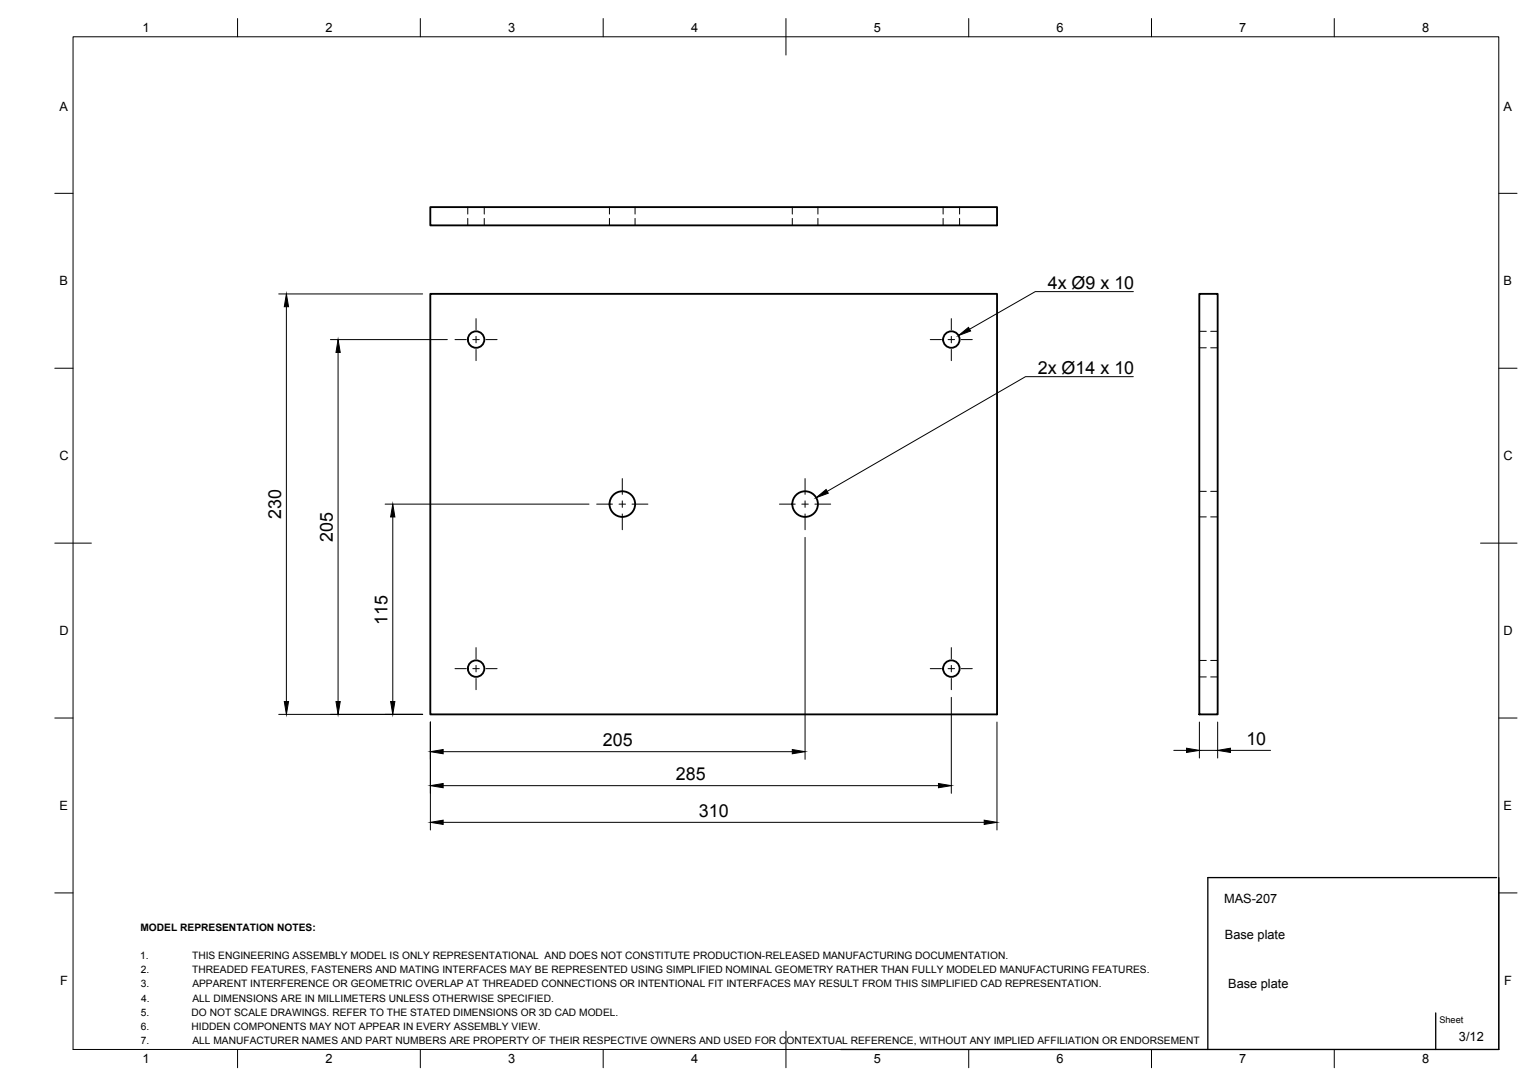
ISO-10303-21;
HEADER;
/* Generated by software containing ST-Developer
 * from STEP Tools, Inc. (www.steptools.com) 
 */

FILE_DESCRIPTION(
/* description */ ('Independent six-slot Geneva indexer. Center distance100, drive radius
50, 60degree indexing per input revolution with120degree engagement an
d240degree dwell. Native machined concave locking faces and relieved d
isk; replaceable retained drive pin; keyed output shaft. Geometry traj
ectory checks use calculated indexing positions, not a contact-dynamic
s simulation. No load or production rating assigned.'),
/* implementation_level */ '2;1');

FILE_NAME(
/* name */ 'Base plate.step',
/* time_stamp */ '2026-11-09T17:53:22-08:00',
/* author */ (''),
/* organization */ (''),
/* preprocessor_version */ 'ST-DEVELOPER v20.2',
/* originating_system */ 'Autodesk Translation Framework v15.17.0.0',
/* authorisation */ '');

FILE_SCHEMA (('AUTOMOTIVE_DESIGN { 1 0 10303 214 3 1 1 }'));
ENDSEC;

DATA;
#10=MECHANICAL_DESIGN_GEOMETRIC_PRESENTATION_REPRESENTATION('',(#101),#4149);
#79=SHAPE_REPRESENTATION_RELATIONSHIP('SRR','None',#4196,#90);
#90=ADVANCED_BREP_SHAPE_REPRESENTATION('',(#112),#4138);
#101=STYLED_ITEM('',(#4260),#112);
#112=MANIFOLD_SOLID_BREP('Body1',#2295);
#123=FACE_BOUND('',#385,.T.);
#124=FACE_BOUND('',#386,.T.);
#125=FACE_BOUND('',#387,.T.);
#126=FACE_BOUND('',#388,.T.);
#127=FACE_BOUND('',#389,.T.);
#128=FACE_BOUND('',#390,.T.);
#129=FACE_BOUND('',#392,.T.);
#130=FACE_BOUND('',#393,.T.);
#131=FACE_BOUND('',#394,.T.);
#132=FACE_BOUND('',#395,.T.);
#133=FACE_BOUND('',#396,.T.);
#134=FACE_BOUND('',#397,.T.);
#161=PLANE('',#2448);
#162=PLANE('',#2449);
#163=PLANE('',#2450);
#164=PLANE('',#2451);
#165=PLANE('',#2452);
#166=PLANE('',#2453);
#238=FACE_OUTER_BOUND('',#374,.T.);
#239=FACE_OUTER_BOUND('',#375,.T.);
#240=FACE_OUTER_BOUND('',#376,.T.);
#241=FACE_OUTER_BOUND('',#377,.T.);
#242=FACE_OUTER_BOUND('',#378,.T.);
#243=FACE_OUTER_BOUND('',#379,.T.);
#244=FACE_OUTER_BOUND('',#380,.T.);
#245=FACE_OUTER_BOUND('',#381,.T.);
#246=FACE_OUTER_BOUND('',#382,.T.);
#247=FACE_OUTER_BOUND('',#383,.T.);
#248=FACE_OUTER_BOUND('',#384,.T.);
#249=FACE_OUTER_BOUND('',#391,.T.);
#374=EDGE_LOOP('',(#1508,#1509,#1510,#1511));
#375=EDGE_LOOP('',(#1512,#1513,#1514,#1515));
#376=EDGE_LOOP('',(#1516,#1517,#1518,#1519));
#377=EDGE_LOOP('',(#1520,#1521,#1522,#1523));
#378=EDGE_LOOP('',(#1524,#1525,#1526,#1527));
#379=EDGE_LOOP('',(#1528,#1529,#1530,#1531));
#380=EDGE_LOOP('',(#1532,#1533,#1534,#1535));
#381=EDGE_LOOP('',(#1536,#1537,#1538,#1539));
#382=EDGE_LOOP('',(#1540,#1541,#1542,#1543));
#383=EDGE_LOOP('',(#1544,#1545,#1546,#1547));
#384=EDGE_LOOP('',(#1548,#1549,#1550,#1551));
#385=EDGE_LOOP('',(#1552));
#386=EDGE_LOOP('',(#1553));
#387=EDGE_LOOP('',(#1554));
#388=EDGE_LOOP('',(#1555));
#389=EDGE_LOOP('',(#1556));
#390=EDGE_LOOP('',(#1557));
#391=EDGE_LOOP('',(#1558,#1559,#1560,#1561));
#392=EDGE_LOOP('',(#1562));
#393=EDGE_LOOP('',(#1563));
#394=EDGE_LOOP('',(#1564));
#395=EDGE_LOOP('',(#1565));
#396=EDGE_LOOP('',(#1566));
#397=EDGE_LOOP('',(#1567));
#548=LINE('',#3473,#720);
#549=LINE('',#3479,#721);
#550=LINE('',#3485,#722);
#551=LINE('',#3491,#723);
#552=LINE('',#3497,#724);
#553=LINE('',#3503,#725);
#554=LINE('',#3508,#726);
#555=LINE('',#3510,#727);
#556=LINE('',#3512,#728);
#557=LINE('',#3513,#729);
#558=LINE('',#3516,#730);
#559=LINE('',#3518,#731);
#560=LINE('',#3519,#732);
#561=LINE('',#3522,#733);
#562=LINE('',#3524,#734);
#563=LINE('',#3525,#735);
#564=LINE('',#3527,#736);
#565=LINE('',#3528,#737);
#720=VECTOR('',#2725,4.5);
#721=VECTOR('',#2732,4.5);
#722=VECTOR('',#2739,4.5);
#723=VECTOR('',#2746,4.5);
#724=VECTOR('',#2753,7.);
#725=VECTOR('',#2760,7.);
#726=VECTOR('',#2765,10.);
#727=VECTOR('',#2766,10.);
#728=VECTOR('',#2767,10.);
#729=VECTOR('',#2768,10.);
#730=VECTOR('',#2771,10.);
#731=VECTOR('',#2772,10.);
#732=VECTOR('',#2773,10.);
#733=VECTOR('',#2776,10.);
#734=VECTOR('',#2777,10.);
#735=VECTOR('',#2778,10.);
#736=VECTOR('',#2781,10.);
#737=VECTOR('',#2782,10.);
#892=CIRCLE('',#2431,4.5);
#893=CIRCLE('',#2432,4.5);
#894=CIRCLE('',#2434,4.5);
#895=CIRCLE('',#2435,4.5);
#896=CIRCLE('',#2437,4.5);
#897=CIRCLE('',#2438,4.5);
#898=CIRCLE('',#2440,4.5);
#899=CIRCLE('',#2441,4.5);
#900=CIRCLE('',#2443,7.);
#901=CIRCLE('',#2444,7.);
#902=CIRCLE('',#2446,7.);
#903=CIRCLE('',#2447,7.);
#1016=VERTEX_POINT('',#3470);
#1017=VERTEX_POINT('',#3472);
#1018=VERTEX_POINT('',#3476);
#1019=VERTEX_POINT('',#3478);
#1020=VERTEX_POINT('',#3482);
#1021=VERTEX_POINT('',#3484);
#1022=VERTEX_POINT('',#3488);
#1023=VERTEX_POINT('',#3490);
#1024=VERTEX_POINT('',#3494);
#1025=VERTEX_POINT('',#3496);
#1026=VERTEX_POINT('',#3500);
#1027=VERTEX_POINT('',#3502);
#1028=VERTEX_POINT('',#3506);
#1029=VERTEX_POINT('',#3507);
#1030=VERTEX_POINT('',#3509);
#1031=VERTEX_POINT('',#3511);
#1032=VERTEX_POINT('',#3515);
#1033=VERTEX_POINT('',#3517);
#1034=VERTEX_POINT('',#3521);
#1035=VERTEX_POINT('',#3523);
#1212=EDGE_CURVE('',#1016,#1016,#892,.T.);
#1213=EDGE_CURVE('',#1016,#1017,#548,.T.);
#1214=EDGE_CURVE('',#1017,#1017,#893,.T.);
#1215=EDGE_CURVE('',#1018,#1018,#894,.T.);
#1216=EDGE_CURVE('',#1018,#1019,#549,.T.);
#1217=EDGE_CURVE('',#1019,#1019,#895,.T.);
#1218=EDGE_CURVE('',#1020,#1020,#896,.T.);
#1219=EDGE_CURVE('',#1020,#1021,#550,.T.);
#1220=EDGE_CURVE('',#1021,#1021,#897,.T.);
#1221=EDGE_CURVE('',#1022,#1022,#898,.T.);
#1222=EDGE_CURVE('',#1022,#1023,#551,.T.);
#1223=EDGE_CURVE('',#1023,#1023,#899,.T.);
#1224=EDGE_CURVE('',#1024,#1024,#900,.T.);
#1225=EDGE_CURVE('',#1024,#1025,#552,.T.);
#1226=EDGE_CURVE('',#1025,#1025,#901,.T.);
#1227=EDGE_CURVE('',#1026,#1026,#902,.T.);
#1228=EDGE_CURVE('',#1026,#1027,#553,.T.);
#1229=EDGE_CURVE('',#1027,#1027,#903,.T.);
#1230=EDGE_CURVE('',#1028,#1029,#554,.F.);
#1231=EDGE_CURVE('',#1029,#1030,#555,.F.);
#1232=EDGE_CURVE('',#1031,#1030,#556,.F.);
#1233=EDGE_CURVE('',#1028,#1031,#557,.F.);
#1234=EDGE_CURVE('',#1032,#1028,#558,.F.);
#1235=EDGE_CURVE('',#1033,#1031,#559,.F.);
#1236=EDGE_CURVE('',#1032,#1033,#560,.F.);
#1237=EDGE_CURVE('',#1034,#1032,#561,.F.);
#1238=EDGE_CURVE('',#1035,#1033,#562,.F.);
#1239=EDGE_CURVE('',#1034,#1035,#563,.T.);
#1240=EDGE_CURVE('',#1029,#1034,#564,.F.);
#1241=EDGE_CURVE('',#1030,#1035,#565,.F.);
#1508=ORIENTED_EDGE('',*,*,#1212,.F.);
#1509=ORIENTED_EDGE('',*,*,#1213,.T.);
#1510=ORIENTED_EDGE('',*,*,#1214,.F.);
#1511=ORIENTED_EDGE('',*,*,#1213,.F.);
#1512=ORIENTED_EDGE('',*,*,#1215,.F.);
#1513=ORIENTED_EDGE('',*,*,#1216,.T.);
#1514=ORIENTED_EDGE('',*,*,#1217,.F.);
#1515=ORIENTED_EDGE('',*,*,#1216,.F.);
#1516=ORIENTED_EDGE('',*,*,#1218,.F.);
#1517=ORIENTED_EDGE('',*,*,#1219,.T.);
#1518=ORIENTED_EDGE('',*,*,#1220,.F.);
#1519=ORIENTED_EDGE('',*,*,#1219,.F.);
#1520=ORIENTED_EDGE('',*,*,#1221,.F.);
#1521=ORIENTED_EDGE('',*,*,#1222,.T.);
#1522=ORIENTED_EDGE('',*,*,#1223,.F.);
#1523=ORIENTED_EDGE('',*,*,#1222,.F.);
#1524=ORIENTED_EDGE('',*,*,#1224,.F.);
#1525=ORIENTED_EDGE('',*,*,#1225,.T.);
#1526=ORIENTED_EDGE('',*,*,#1226,.F.);
#1527=ORIENTED_EDGE('',*,*,#1225,.F.);
#1528=ORIENTED_EDGE('',*,*,#1227,.F.);
#1529=ORIENTED_EDGE('',*,*,#1228,.T.);
#1530=ORIENTED_EDGE('',*,*,#1229,.F.);
#1531=ORIENTED_EDGE('',*,*,#1228,.F.);
#1532=ORIENTED_EDGE('',*,*,#1230,.T.);
#1533=ORIENTED_EDGE('',*,*,#1231,.T.);
#1534=ORIENTED_EDGE('',*,*,#1232,.F.);
#1535=ORIENTED_EDGE('',*,*,#1233,.F.);
#1536=ORIENTED_EDGE('',*,*,#1234,.T.);
#1537=ORIENTED_EDGE('',*,*,#1233,.T.);
#1538=ORIENTED_EDGE('',*,*,#1235,.F.);
#1539=ORIENTED_EDGE('',*,*,#1236,.F.);
#1540=ORIENTED_EDGE('',*,*,#1237,.T.);
#1541=ORIENTED_EDGE('',*,*,#1236,.T.);
#1542=ORIENTED_EDGE('',*,*,#1238,.F.);
#1543=ORIENTED_EDGE('',*,*,#1239,.F.);
#1544=ORIENTED_EDGE('',*,*,#1240,.T.);
#1545=ORIENTED_EDGE('',*,*,#1239,.T.);
#1546=ORIENTED_EDGE('',*,*,#1241,.F.);
#1547=ORIENTED_EDGE('',*,*,#1231,.F.);
#1548=ORIENTED_EDGE('',*,*,#1241,.T.);
#1549=ORIENTED_EDGE('',*,*,#1238,.T.);
#1550=ORIENTED_EDGE('',*,*,#1235,.T.);
#1551=ORIENTED_EDGE('',*,*,#1232,.T.);
#1552=ORIENTED_EDGE('',*,*,#1227,.T.);
#1553=ORIENTED_EDGE('',*,*,#1224,.T.);
#1554=ORIENTED_EDGE('',*,*,#1221,.T.);
#1555=ORIENTED_EDGE('',*,*,#1218,.T.);
#1556=ORIENTED_EDGE('',*,*,#1215,.T.);
#1557=ORIENTED_EDGE('',*,*,#1212,.T.);
#1558=ORIENTED_EDGE('',*,*,#1240,.F.);
#1559=ORIENTED_EDGE('',*,*,#1230,.F.);
#1560=ORIENTED_EDGE('',*,*,#1234,.F.);
#1561=ORIENTED_EDGE('',*,*,#1237,.F.);
#1562=ORIENTED_EDGE('',*,*,#1229,.T.);
#1563=ORIENTED_EDGE('',*,*,#1226,.T.);
#1564=ORIENTED_EDGE('',*,*,#1223,.T.);
#1565=ORIENTED_EDGE('',*,*,#1220,.T.);
#1566=ORIENTED_EDGE('',*,*,#1217,.T.);
#1567=ORIENTED_EDGE('',*,*,#1214,.T.);
#2100=CYLINDRICAL_SURFACE('',#2430,4.5);
#2101=CYLINDRICAL_SURFACE('',#2433,4.5);
#2102=CYLINDRICAL_SURFACE('',#2436,4.5);
#2103=CYLINDRICAL_SURFACE('',#2439,4.5);
#2104=CYLINDRICAL_SURFACE('',#2442,7.);
#2105=CYLINDRICAL_SURFACE('',#2445,7.);
#2159=ADVANCED_FACE('',(#238),#2100,.F.);
#2160=ADVANCED_FACE('',(#239),#2101,.F.);
#2161=ADVANCED_FACE('',(#240),#2102,.F.);
#2162=ADVANCED_FACE('',(#241),#2103,.F.);
#2163=ADVANCED_FACE('',(#242),#2104,.F.);
#2164=ADVANCED_FACE('',(#243),#2105,.F.);
#2165=ADVANCED_FACE('',(#244),#161,.T.);
#2166=ADVANCED_FACE('',(#245),#162,.T.);
#2167=ADVANCED_FACE('',(#246),#163,.T.);
#2168=ADVANCED_FACE('',(#247),#164,.T.);
#2169=ADVANCED_FACE('',(#248,#123,#124,#125,#126,#127,#128),#165,.T.);
#2170=ADVANCED_FACE('',(#249,#129,#130,#131,#132,#133,#134),#166,.F.);
#2295=CLOSED_SHELL('',(#2159,#2160,#2161,#2162,#2163,#2164,#2165,#2166,
#2167,#2168,#2169,#2170));
#2429=AXIS2_PLACEMENT_3D('',#3468,#2719,#2720);
#2430=AXIS2_PLACEMENT_3D('',#3469,#2721,#2722);
#2431=AXIS2_PLACEMENT_3D('',#3471,#2723,#2724);
#2432=AXIS2_PLACEMENT_3D('',#3474,#2726,#2727);
#2433=AXIS2_PLACEMENT_3D('',#3475,#2728,#2729);
#2434=AXIS2_PLACEMENT_3D('',#3477,#2730,#2731);
#2435=AXIS2_PLACEMENT_3D('',#3480,#2733,#2734);
#2436=AXIS2_PLACEMENT_3D('',#3481,#2735,#2736);
#2437=AXIS2_PLACEMENT_3D('',#3483,#2737,#2738);
#2438=AXIS2_PLACEMENT_3D('',#3486,#2740,#2741);
#2439=AXIS2_PLACEMENT_3D('',#3487,#2742,#2743);
#2440=AXIS2_PLACEMENT_3D('',#3489,#2744,#2745);
#2441=AXIS2_PLACEMENT_3D('',#3492,#2747,#2748);
#2442=AXIS2_PLACEMENT_3D('',#3493,#2749,#2750);
#2443=AXIS2_PLACEMENT_3D('',#3495,#2751,#2752);
#2444=AXIS2_PLACEMENT_3D('',#3498,#2754,#2755);
#2445=AXIS2_PLACEMENT_3D('',#3499,#2756,#2757);
#2446=AXIS2_PLACEMENT_3D('',#3501,#2758,#2759);
#2447=AXIS2_PLACEMENT_3D('',#3504,#2761,#2762);
#2448=AXIS2_PLACEMENT_3D('',#3505,#2763,#2764);
#2449=AXIS2_PLACEMENT_3D('',#3514,#2769,#2770);
#2450=AXIS2_PLACEMENT_3D('',#3520,#2774,#2775);
#2451=AXIS2_PLACEMENT_3D('',#3526,#2779,#2780);
#2452=AXIS2_PLACEMENT_3D('',#3529,#2783,#2784);
#2453=AXIS2_PLACEMENT_3D('',#3530,#2785,#2786);
#2719=DIRECTION('axis',(0.,0.,1.));
#2720=DIRECTION('refdir',(1.,0.,0.));
#2721=DIRECTION('center_axis',(0.,0.,-1.));
#2722=DIRECTION('ref_axis',(1.,0.,0.));
#2723=DIRECTION('center_axis',(0.,0.,-1.));
#2724=DIRECTION('ref_axis',(1.,0.,0.));
#2725=DIRECTION('',(0.,0.,-1.));
#2726=DIRECTION('center_axis',(0.,0.,1.));
#2727=DIRECTION('ref_axis',(1.,0.,0.));
#2728=DIRECTION('center_axis',(0.,0.,-1.));
#2729=DIRECTION('ref_axis',(1.,0.,0.));
#2730=DIRECTION('center_axis',(0.,0.,-1.));
#2731=DIRECTION('ref_axis',(1.,0.,0.));
#2732=DIRECTION('',(0.,0.,-1.));
#2733=DIRECTION('center_axis',(0.,0.,1.));
#2734=DIRECTION('ref_axis',(1.,0.,0.));
#2735=DIRECTION('center_axis',(0.,0.,-1.));
#2736=DIRECTION('ref_axis',(1.,0.,0.));
#2737=DIRECTION('center_axis',(0.,0.,-1.));
#2738=DIRECTION('ref_axis',(1.,0.,0.));
#2739=DIRECTION('',(0.,0.,-1.));
#2740=DIRECTION('center_axis',(0.,0.,1.));
#2741=DIRECTION('ref_axis',(1.,0.,0.));
#2742=DIRECTION('center_axis',(0.,0.,-1.));
#2743=DIRECTION('ref_axis',(1.,0.,0.));
#2744=DIRECTION('center_axis',(0.,0.,-1.));
#2745=DIRECTION('ref_axis',(1.,0.,0.));
#2746=DIRECTION('',(0.,0.,-1.));
#2747=DIRECTION('center_axis',(0.,0.,1.));
#2748=DIRECTION('ref_axis',(1.,0.,0.));
#2749=DIRECTION('center_axis',(0.,0.,-1.));
#2750=DIRECTION('ref_axis',(1.,0.,0.));
#2751=DIRECTION('center_axis',(0.,0.,-1.));
#2752=DIRECTION('ref_axis',(1.,0.,0.));
#2753=DIRECTION('',(0.,0.,-1.));
#2754=DIRECTION('center_axis',(0.,0.,1.));
#2755=DIRECTION('ref_axis',(1.,0.,0.));
#2756=DIRECTION('center_axis',(0.,0.,-1.));
#2757=DIRECTION('ref_axis',(1.,0.,0.));
#2758=DIRECTION('center_axis',(0.,0.,-1.));
#2759=DIRECTION('ref_axis',(1.,0.,0.));
#2760=DIRECTION('',(0.,0.,-1.));
#2761=DIRECTION('center_axis',(0.,0.,1.));
#2762=DIRECTION('ref_axis',(1.,0.,0.));
#2763=DIRECTION('center_axis',(0.,1.,0.));
#2764=DIRECTION('ref_axis',(-1.,0.,0.));
#2765=DIRECTION('',(1.,0.,0.));
#2766=DIRECTION('',(0.,0.,-1.));
#2767=DIRECTION('',(1.,0.,0.));
#2768=DIRECTION('',(0.,0.,-1.));
#2769=DIRECTION('center_axis',(1.,0.,0.));
#2770=DIRECTION('ref_axis',(0.,1.,0.));
#2771=DIRECTION('',(0.,-1.,0.));
#2772=DIRECTION('',(0.,-1.,0.));
#2773=DIRECTION('',(0.,0.,-1.));
#2774=DIRECTION('center_axis',(0.,-1.,0.));
#2775=DIRECTION('ref_axis',(1.,0.,0.));
#2776=DIRECTION('',(-1.,0.,0.));
#2777=DIRECTION('',(-1.,0.,0.));
#2778=DIRECTION('',(0.,0.,1.));
#2779=DIRECTION('center_axis',(-1.,0.,0.));
#2780=DIRECTION('ref_axis',(0.,-1.,0.));
#2781=DIRECTION('',(0.,1.,0.));
#2782=DIRECTION('',(0.,1.,0.));
#2783=DIRECTION('center_axis',(0.,0.,1.));
#2784=DIRECTION('ref_axis',(1.,0.,0.));
#2785=DIRECTION('center_axis',(0.,0.,1.));
#2786=DIRECTION('ref_axis',(1.,0.,0.));
#3468=CARTESIAN_POINT('',(0.,0.,0.));
#3469=CARTESIAN_POINT('Origin',(180.,-90.,5.));
#3470=CARTESIAN_POINT('',(175.5,-90.,10.));
#3471=CARTESIAN_POINT('Origin',(180.,-90.,10.));
#3472=CARTESIAN_POINT('',(175.5,-90.,0.));
#3473=CARTESIAN_POINT('',(175.5,-90.,5.));
#3474=CARTESIAN_POINT('Origin',(180.,-90.,0.));
#3475=CARTESIAN_POINT('Origin',(-80.,-90.,5.));
#3476=CARTESIAN_POINT('',(-84.5,-90.,10.));
#3477=CARTESIAN_POINT('Origin',(-80.,-90.,10.));
#3478=CARTESIAN_POINT('',(-84.5,-90.,0.));
#3479=CARTESIAN_POINT('',(-84.5,-90.,5.));
#3480=CARTESIAN_POINT('Origin',(-80.,-90.,0.));
#3481=CARTESIAN_POINT('Origin',(-80.,90.,5.));
#3482=CARTESIAN_POINT('',(-84.5,90.,10.));
#3483=CARTESIAN_POINT('Origin',(-80.,90.,10.));
#3484=CARTESIAN_POINT('',(-84.5,90.,0.));
#3485=CARTESIAN_POINT('',(-84.5,90.,5.));
#3486=CARTESIAN_POINT('Origin',(-80.,90.,0.));
#3487=CARTESIAN_POINT('Origin',(180.,90.,5.));
#3488=CARTESIAN_POINT('',(175.5,90.,10.));
#3489=CARTESIAN_POINT('Origin',(180.,90.,10.));
#3490=CARTESIAN_POINT('',(175.5,90.,0.));
#3491=CARTESIAN_POINT('',(175.5,90.,5.));
#3492=CARTESIAN_POINT('Origin',(180.,90.,0.));
#3493=CARTESIAN_POINT('Origin',(0.,0.,5.));
#3494=CARTESIAN_POINT('',(-7.,8.57252759403147E-16,10.));
#3495=CARTESIAN_POINT('Origin',(0.,0.,10.));
#3496=CARTESIAN_POINT('',(-7.,8.57252759403147E-16,0.));
#3497=CARTESIAN_POINT('',(-7.,8.57252759403147E-16,5.));
#3498=CARTESIAN_POINT('Origin',(0.,0.,0.));
#3499=CARTESIAN_POINT('Origin',(100.,0.,5.));
#3500=CARTESIAN_POINT('',(93.,8.57252759403147E-16,10.));
#3501=CARTESIAN_POINT('Origin',(100.,0.,10.));
#3502=CARTESIAN_POINT('',(93.,8.57252759403147E-16,0.));
#3503=CARTESIAN_POINT('',(93.,8.57252759403147E-16,5.));
#3504=CARTESIAN_POINT('Origin',(100.,0.,0.));
#3505=CARTESIAN_POINT('Origin',(200.,115.,0.));
#3506=CARTESIAN_POINT('',(205.,115.,0.));
#3507=CARTESIAN_POINT('',(-105.,115.,0.));
#3508=CARTESIAN_POINT('',(125.,115.,0.));
#3509=CARTESIAN_POINT('',(-105.,115.,10.));
#3510=CARTESIAN_POINT('',(-105.,115.,0.));
#3511=CARTESIAN_POINT('',(205.,115.,10.));
#3512=CARTESIAN_POINT('',(125.,115.,10.));
#3513=CARTESIAN_POINT('',(205.,115.,0.));
#3514=CARTESIAN_POINT('Origin',(205.,-110.,0.));
#3515=CARTESIAN_POINT('',(205.,-115.,0.));
#3516=CARTESIAN_POINT('',(205.,-55.,0.));
#3517=CARTESIAN_POINT('',(205.,-115.,10.));
#3518=CARTESIAN_POINT('',(205.,-55.,10.));
#3519=CARTESIAN_POINT('',(205.,-115.,0.));
#3520=CARTESIAN_POINT('Origin',(-100.,-115.,0.));
#3521=CARTESIAN_POINT('',(-105.,-115.,0.));
#3522=CARTESIAN_POINT('',(-25.,-115.,0.));
#3523=CARTESIAN_POINT('',(-105.,-115.,10.));
#3524=CARTESIAN_POINT('',(-25.,-115.,10.));
#3525=CARTESIAN_POINT('',(-105.,-115.,0.));
#3526=CARTESIAN_POINT('Origin',(-105.,110.,0.));
#3527=CARTESIAN_POINT('',(-105.,55.,0.));
#3528=CARTESIAN_POINT('',(-105.,55.,10.));
#3529=CARTESIAN_POINT('Origin',(50.,0.,10.));
#3530=CARTESIAN_POINT('Origin',(50.,0.,0.));
#4125=UNCERTAINTY_MEASURE_WITH_UNIT(LENGTH_MEASURE(0.01),#4150,
'DISTANCE_ACCURACY_VALUE',
'Maximum model space distance between geometric entities at asserted c
onnectivities');
#4136=UNCERTAINTY_MEASURE_WITH_UNIT(LENGTH_MEASURE(0.01),#4150,
'DISTANCE_ACCURACY_VALUE',
'Maximum model space distance between geometric entities at asserted c
onnectivities');
#4138=(
GEOMETRIC_REPRESENTATION_CONTEXT(3)
GLOBAL_UNCERTAINTY_ASSIGNED_CONTEXT((#4125))
GLOBAL_UNIT_ASSIGNED_CONTEXT((#4150,#4152,#4153))
REPRESENTATION_CONTEXT('','3D')
);
#4149=(
GEOMETRIC_REPRESENTATION_CONTEXT(3)
GLOBAL_UNCERTAINTY_ASSIGNED_CONTEXT((#4136))
GLOBAL_UNIT_ASSIGNED_CONTEXT((#4150,#4152,#4153))
REPRESENTATION_CONTEXT('','3D')
);
#4150=(
LENGTH_UNIT()
NAMED_UNIT(*)
SI_UNIT(.MILLI.,.METRE.)
);
#4152=(
NAMED_UNIT(*)
PLANE_ANGLE_UNIT()
SI_UNIT($,.RADIAN.)
);
#4153=(
NAMED_UNIT(*)
SI_UNIT($,.STERADIAN.)
SOLID_ANGLE_UNIT()
);
#4155=SHAPE_DEFINITION_REPRESENTATION(#4167,#4196);
#4167=PRODUCT_DEFINITION_SHAPE('',$,#4209);
#4196=SHAPE_REPRESENTATION('',(#2429),#4138);
#4207=PRODUCT_DEFINITION_CONTEXT('part definition',#4245,'design');
#4209=PRODUCT_DEFINITION('Base plate','Base plate',#4221,#4207);
#4221=PRODUCT_DEFINITION_FORMATION('',$,#4248);
#4245=APPLICATION_CONTEXT(
'Core Data for Automotive Mechanical Design Process');
#4246=PRODUCT_CONTEXT('part definition',#4245,'mechanical');
#4248=PRODUCT('Base plate','Base plate','Base plate',(#4246));
#4260=PRESENTATION_STYLE_ASSIGNMENT((#4270));
#4270=SURFACE_STYLE_USAGE(.BOTH.,#4280);
#4280=SURFACE_SIDE_STYLE('',(#4290));
#4290=SURFACE_STYLE_FILL_AREA(#4300);
#4300=FILL_AREA_STYLE('Base gray',(#4310));
#4310=FILL_AREA_STYLE_COLOUR('Base gray',#4320);
#4320=COLOUR_RGB('Base gray',0.407843137254902,0.447058823529412,0.498039215686275);
ENDSEC;
END-ISO-10303-21;
